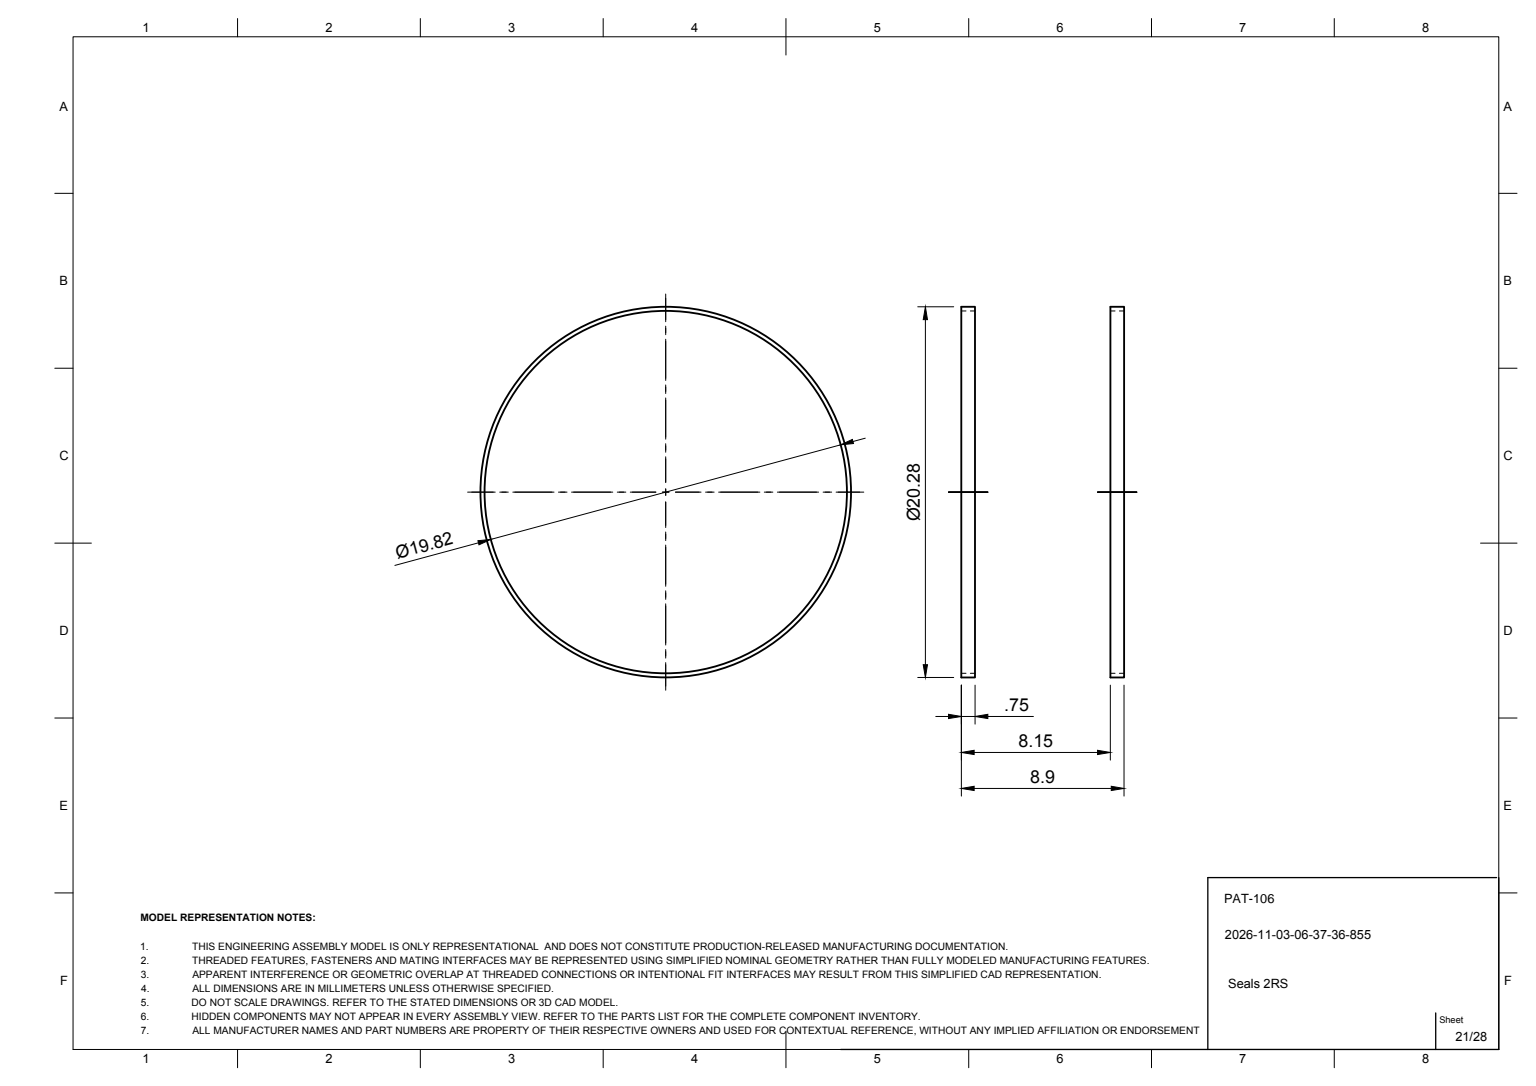
ISO-10303-21;
HEADER;
/* Generated by software containing ST-Developer
 * from STEP Tools, Inc. (www.steptools.com) 
 */

FILE_DESCRIPTION(
/* description */ ('Torsion-spring ratchet demonstrator'),
/* implementation_level */ '2;1');

FILE_NAME(
/* name */ 'Seals 2RS.step',
/* time_stamp */ '2026-10-29T17:29:17-07:00',
/* author */ (''),
/* organization */ (''),
/* preprocessor_version */ 'ST-DEVELOPER v20.2',
/* originating_system */ 'Autodesk Translation Framework v15.17.0.0',
/* authorisation */ '');

FILE_SCHEMA (('AUTOMOTIVE_DESIGN { 1 0 10303 214 3 1 1 }'));
ENDSEC;

DATA;
#10=MECHANICAL_DESIGN_GEOMETRIC_PRESENTATION_REPRESENTATION('',(#303,#304),#11258);
#248=SHAPE_REPRESENTATION_RELATIONSHIP('SRR','None',#11375,#272);
#272=ADVANCED_BREP_SHAPE_REPRESENTATION('',(#335,#336),#11245);
#303=STYLED_ITEM('',(#11584),#335);
#304=STYLED_ITEM('',(#11584),#336);
#335=MANIFOLD_SOLID_BREP('Body1',#5174);
#336=MANIFOLD_SOLID_BREP('Body2',#5175);
#414=FACE_BOUND('',#1145,.T.);
#415=FACE_BOUND('',#1148,.T.);
#416=FACE_BOUND('',#1151,.T.);
#417=FACE_BOUND('',#1154,.T.);
#502=PLANE('',#5793);
#503=PLANE('',#5798);
#504=PLANE('',#5801);
#505=PLANE('',#5806);
#770=FACE_OUTER_BOUND('',#1144,.T.);
#771=FACE_OUTER_BOUND('',#1146,.T.);
#772=FACE_OUTER_BOUND('',#1147,.T.);
#773=FACE_OUTER_BOUND('',#1149,.T.);
#774=FACE_OUTER_BOUND('',#1150,.T.);
#775=FACE_OUTER_BOUND('',#1152,.T.);
#776=FACE_OUTER_BOUND('',#1153,.T.);
#777=FACE_OUTER_BOUND('',#1155,.T.);
#1144=EDGE_LOOP('',(#4050));
#1145=EDGE_LOOP('',(#4051));
#1146=EDGE_LOOP('',(#4052,#4053,#4054,#4055));
#1147=EDGE_LOOP('',(#4056));
#1148=EDGE_LOOP('',(#4057));
#1149=EDGE_LOOP('',(#4058,#4059,#4060,#4061));
#1150=EDGE_LOOP('',(#4062));
#1151=EDGE_LOOP('',(#4063));
#1152=EDGE_LOOP('',(#4064,#4065,#4066,#4067));
#1153=EDGE_LOOP('',(#4068));
#1154=EDGE_LOOP('',(#4069));
#1155=EDGE_LOOP('',(#4070,#4071,#4072,#4073));
#1431=LINE('',#8769,#1814);
#1432=LINE('',#8774,#1815);
#1433=LINE('',#8783,#1816);
#1434=LINE('',#8788,#1817);
#1814=VECTOR('',#6862,1.013815);
#1815=VECTOR('',#6869,0.991185);
#1816=VECTOR('',#6880,1.013815);
#1817=VECTOR('',#6887,0.991185);
#2267=CIRCLE('',#5794,1.013815);
#2268=CIRCLE('',#5795,0.991185);
#2269=CIRCLE('',#5797,1.013815);
#2270=CIRCLE('',#5799,0.991185);
#2271=CIRCLE('',#5802,1.013815);
#2272=CIRCLE('',#5803,0.991185);
#2273=CIRCLE('',#5805,1.013815);
#2274=CIRCLE('',#5807,0.991185);
#2547=VERTEX_POINT('',#8762);
#2548=VERTEX_POINT('',#8764);
#2549=VERTEX_POINT('',#8767);
#2550=VERTEX_POINT('',#8771);
#2551=VERTEX_POINT('',#8776);
#2552=VERTEX_POINT('',#8778);
#2553=VERTEX_POINT('',#8781);
#2554=VERTEX_POINT('',#8785);
#3085=EDGE_CURVE('',#2547,#2547,#2267,.T.);
#3086=EDGE_CURVE('',#2548,#2548,#2268,.T.);
#3087=EDGE_CURVE('',#2549,#2549,#2269,.T.);
#3088=EDGE_CURVE('',#2549,#2547,#1431,.T.);
#3089=EDGE_CURVE('',#2550,#2550,#2270,.T.);
#3090=EDGE_CURVE('',#2550,#2548,#1432,.T.);
#3091=EDGE_CURVE('',#2551,#2551,#2271,.T.);
#3092=EDGE_CURVE('',#2552,#2552,#2272,.T.);
#3093=EDGE_CURVE('',#2553,#2553,#2273,.T.);
#3094=EDGE_CURVE('',#2553,#2551,#1433,.T.);
#3095=EDGE_CURVE('',#2554,#2554,#2274,.T.);
#3096=EDGE_CURVE('',#2554,#2552,#1434,.T.);
#4050=ORIENTED_EDGE('',*,*,#3085,.F.);
#4051=ORIENTED_EDGE('',*,*,#3086,.T.);
#4052=ORIENTED_EDGE('',*,*,#3087,.F.);
#4053=ORIENTED_EDGE('',*,*,#3088,.T.);
#4054=ORIENTED_EDGE('',*,*,#3085,.T.);
#4055=ORIENTED_EDGE('',*,*,#3088,.F.);
#4056=ORIENTED_EDGE('',*,*,#3087,.T.);
#4057=ORIENTED_EDGE('',*,*,#3089,.F.);
#4058=ORIENTED_EDGE('',*,*,#3089,.T.);
#4059=ORIENTED_EDGE('',*,*,#3090,.T.);
#4060=ORIENTED_EDGE('',*,*,#3086,.F.);
#4061=ORIENTED_EDGE('',*,*,#3090,.F.);
#4062=ORIENTED_EDGE('',*,*,#3091,.F.);
#4063=ORIENTED_EDGE('',*,*,#3092,.T.);
#4064=ORIENTED_EDGE('',*,*,#3093,.F.);
#4065=ORIENTED_EDGE('',*,*,#3094,.T.);
#4066=ORIENTED_EDGE('',*,*,#3091,.T.);
#4067=ORIENTED_EDGE('',*,*,#3094,.F.);
#4068=ORIENTED_EDGE('',*,*,#3093,.T.);
#4069=ORIENTED_EDGE('',*,*,#3095,.F.);
#4070=ORIENTED_EDGE('',*,*,#3095,.T.);
#4071=ORIENTED_EDGE('',*,*,#3096,.T.);
#4072=ORIENTED_EDGE('',*,*,#3092,.F.);
#4073=ORIENTED_EDGE('',*,*,#3096,.F.);
#4824=CYLINDRICAL_SURFACE('',#5796,1.013815);
#4825=CYLINDRICAL_SURFACE('',#5800,0.991185);
#4826=CYLINDRICAL_SURFACE('',#5804,1.013815);
#4827=CYLINDRICAL_SURFACE('',#5808,0.991185);
#4996=ADVANCED_FACE('',(#770,#414),#502,.T.);
#4997=ADVANCED_FACE('',(#771),#4824,.T.);
#4998=ADVANCED_FACE('',(#772,#415),#503,.T.);
#4999=ADVANCED_FACE('',(#773),#4825,.F.);
#5000=ADVANCED_FACE('',(#774,#416),#504,.T.);
#5001=ADVANCED_FACE('',(#775),#4826,.T.);
#5002=ADVANCED_FACE('',(#776,#417),#505,.T.);
#5003=ADVANCED_FACE('',(#777),#4827,.F.);
#5174=CLOSED_SHELL('',(#4996,#4997,#4998,#4999));
#5175=CLOSED_SHELL('',(#5000,#5001,#5002,#5003));
#5792=AXIS2_PLACEMENT_3D('',#8760,#6850,#6851);
#5793=AXIS2_PLACEMENT_3D('',#8761,#6852,#6853);
#5794=AXIS2_PLACEMENT_3D('',#8763,#6854,#6855);
#5795=AXIS2_PLACEMENT_3D('',#8765,#6856,#6857);
#5796=AXIS2_PLACEMENT_3D('',#8766,#6858,#6859);
#5797=AXIS2_PLACEMENT_3D('',#8768,#6860,#6861);
#5798=AXIS2_PLACEMENT_3D('',#8770,#6863,#6864);
#5799=AXIS2_PLACEMENT_3D('',#8772,#6865,#6866);
#5800=AXIS2_PLACEMENT_3D('',#8773,#6867,#6868);
#5801=AXIS2_PLACEMENT_3D('',#8775,#6870,#6871);
#5802=AXIS2_PLACEMENT_3D('',#8777,#6872,#6873);
#5803=AXIS2_PLACEMENT_3D('',#8779,#6874,#6875);
#5804=AXIS2_PLACEMENT_3D('',#8780,#6876,#6877);
#5805=AXIS2_PLACEMENT_3D('',#8782,#6878,#6879);
#5806=AXIS2_PLACEMENT_3D('',#8784,#6881,#6882);
#5807=AXIS2_PLACEMENT_3D('',#8786,#6883,#6884);
#5808=AXIS2_PLACEMENT_3D('',#8787,#6885,#6886);
#6850=DIRECTION('axis',(0.,0.,1.));
#6851=DIRECTION('refdir',(1.,0.,0.));
#6852=DIRECTION('center_axis',(0.,1.,0.));
#6853=DIRECTION('ref_axis',(0.,0.,1.));
#6854=DIRECTION('center_axis',(0.,-1.,0.));
#6855=DIRECTION('ref_axis',(1.,0.,0.));
#6856=DIRECTION('center_axis',(0.,-1.,0.));
#6857=DIRECTION('ref_axis',(1.,0.,0.));
#6858=DIRECTION('center_axis',(0.,-1.,0.));
#6859=DIRECTION('ref_axis',(1.,0.,0.));
#6860=DIRECTION('center_axis',(0.,-1.,0.));
#6861=DIRECTION('ref_axis',(1.,0.,0.));
#6862=DIRECTION('',(0.,1.,0.));
#6863=DIRECTION('center_axis',(0.,-1.,0.));
#6864=DIRECTION('ref_axis',(0.,0.,-1.));
#6865=DIRECTION('center_axis',(0.,-1.,0.));
#6866=DIRECTION('ref_axis',(1.,0.,0.));
#6867=DIRECTION('center_axis',(0.,-1.,0.));
#6868=DIRECTION('ref_axis',(1.,0.,0.));
#6869=DIRECTION('',(0.,1.,0.));
#6870=DIRECTION('center_axis',(0.,1.,0.));
#6871=DIRECTION('ref_axis',(0.,0.,1.));
#6872=DIRECTION('center_axis',(0.,-1.,0.));
#6873=DIRECTION('ref_axis',(1.,0.,0.));
#6874=DIRECTION('center_axis',(0.,-1.,0.));
#6875=DIRECTION('ref_axis',(1.,0.,0.));
#6876=DIRECTION('center_axis',(0.,-1.,0.));
#6877=DIRECTION('ref_axis',(1.,0.,0.));
#6878=DIRECTION('center_axis',(0.,-1.,0.));
#6879=DIRECTION('ref_axis',(1.,0.,0.));
#6880=DIRECTION('',(0.,1.,0.));
#6881=DIRECTION('center_axis',(0.,-1.,0.));
#6882=DIRECTION('ref_axis',(0.,0.,-1.));
#6883=DIRECTION('center_axis',(0.,-1.,0.));
#6884=DIRECTION('ref_axis',(1.,0.,0.));
#6885=DIRECTION('center_axis',(0.,-1.,0.));
#6886=DIRECTION('ref_axis',(1.,0.,0.));
#6887=DIRECTION('',(0.,1.,0.));
#8760=CARTESIAN_POINT('',(0.,0.,0.));
#8761=CARTESIAN_POINT('Origin',(1.013815,0.445,0.));
#8762=CARTESIAN_POINT('',(-1.013815,0.445,-1.24156529467757E-16));
#8763=CARTESIAN_POINT('Origin',(0.,0.445,0.));
#8764=CARTESIAN_POINT('',(-0.991185,0.445,-1.21385153761287E-16));
#8765=CARTESIAN_POINT('Origin',(0.,0.445,0.));
#8766=CARTESIAN_POINT('Origin',(0.,0.4075,0.));
#8767=CARTESIAN_POINT('',(-1.013815,0.37,-1.24156529467757E-16));
#8768=CARTESIAN_POINT('Origin',(0.,0.37,0.));
#8769=CARTESIAN_POINT('',(-1.013815,0.4075,-1.24156529467757E-16));
#8770=CARTESIAN_POINT('Origin',(0.991185,0.37,0.));
#8771=CARTESIAN_POINT('',(-0.991185,0.37,-1.21385153761287E-16));
#8772=CARTESIAN_POINT('Origin',(0.,0.37,0.));
#8773=CARTESIAN_POINT('Origin',(0.,0.4075,0.));
#8774=CARTESIAN_POINT('',(-0.991185,0.4075,-1.21385153761287E-16));
#8775=CARTESIAN_POINT('Origin',(1.013815,-0.37,0.));
#8776=CARTESIAN_POINT('',(-1.013815,-0.37,-1.24156529467757E-16));
#8777=CARTESIAN_POINT('Origin',(0.,-0.37,0.));
#8778=CARTESIAN_POINT('',(-0.991185,-0.37,-1.21385153761287E-16));
#8779=CARTESIAN_POINT('Origin',(0.,-0.37,0.));
#8780=CARTESIAN_POINT('Origin',(0.,-0.4075,0.));
#8781=CARTESIAN_POINT('',(-1.013815,-0.445,-1.24156529467757E-16));
#8782=CARTESIAN_POINT('Origin',(0.,-0.445,0.));
#8783=CARTESIAN_POINT('',(-1.013815,-0.4075,-1.24156529467757E-16));
#8784=CARTESIAN_POINT('Origin',(0.991185,-0.445,0.));
#8785=CARTESIAN_POINT('',(-0.991185,-0.445,-1.21385153761287E-16));
#8786=CARTESIAN_POINT('Origin',(0.,-0.445,0.));
#8787=CARTESIAN_POINT('Origin',(0.,-0.4075,0.));
#8788=CARTESIAN_POINT('',(-0.991185,-0.4075,-1.21385153761287E-16));
#11215=UNCERTAINTY_MEASURE_WITH_UNIT(LENGTH_MEASURE(0.001),#11259,
'DISTANCE_ACCURACY_VALUE',
'Maximum model space distance between geometric entities at asserted c
onnectivities');
#11228=UNCERTAINTY_MEASURE_WITH_UNIT(LENGTH_MEASURE(0.001),#11259,
'DISTANCE_ACCURACY_VALUE',
'Maximum model space distance between geometric entities at asserted c
onnectivities');
#11245=(
GEOMETRIC_REPRESENTATION_CONTEXT(3)
GLOBAL_UNCERTAINTY_ASSIGNED_CONTEXT((#11215))
GLOBAL_UNIT_ASSIGNED_CONTEXT((#11259,#11261,#11262))
REPRESENTATION_CONTEXT('','3D')
);
#11258=(
GEOMETRIC_REPRESENTATION_CONTEXT(3)
GLOBAL_UNCERTAINTY_ASSIGNED_CONTEXT((#11228))
GLOBAL_UNIT_ASSIGNED_CONTEXT((#11259,#11261,#11262))
REPRESENTATION_CONTEXT('','3D')
);
#11259=(
LENGTH_UNIT()
NAMED_UNIT(*)
SI_UNIT(.CENTI.,.METRE.)
);
#11261=(
NAMED_UNIT(*)
PLANE_ANGLE_UNIT()
SI_UNIT($,.RADIAN.)
);
#11262=(
NAMED_UNIT(*)
SI_UNIT($,.STERADIAN.)
SOLID_ANGLE_UNIT()
);
#11279=SHAPE_DEFINITION_REPRESENTATION(#11308,#11375);
#11308=PRODUCT_DEFINITION_SHAPE('',$,#11405);
#11375=SHAPE_REPRESENTATION('',(#5792),#11245);
#11388=PRODUCT_DEFINITION_CONTEXT('part definition',#11477,'design');
#11405=PRODUCT_DEFINITION('Seals 2RS','Seals 2RS',#11434,#11388);
#11434=PRODUCT_DEFINITION_FORMATION('',$,#11495);
#11477=APPLICATION_CONTEXT(
'Core Data for Automotive Mechanical Design Process');
#11478=PRODUCT_CONTEXT('part definition',#11477,'mechanical');
#11495=PRODUCT('Seals 2RS','Seals 2RS','Seals 2RS',(#11478));
#11578=COLOUR_RGB('Grey',0.48,0.52,0.57);
#11579=FILL_AREA_STYLE_COLOUR('',#11578);
#11580=FILL_AREA_STYLE('',(#11579));
#11581=SURFACE_STYLE_FILL_AREA(#11580);
#11582=SURFACE_SIDE_STYLE('',(#11581));
#11583=SURFACE_STYLE_USAGE(.BOTH.,#11582);
#11584=PRESENTATION_STYLE_ASSIGNMENT((#11583));
ENDSEC;
END-ISO-10303-21;
